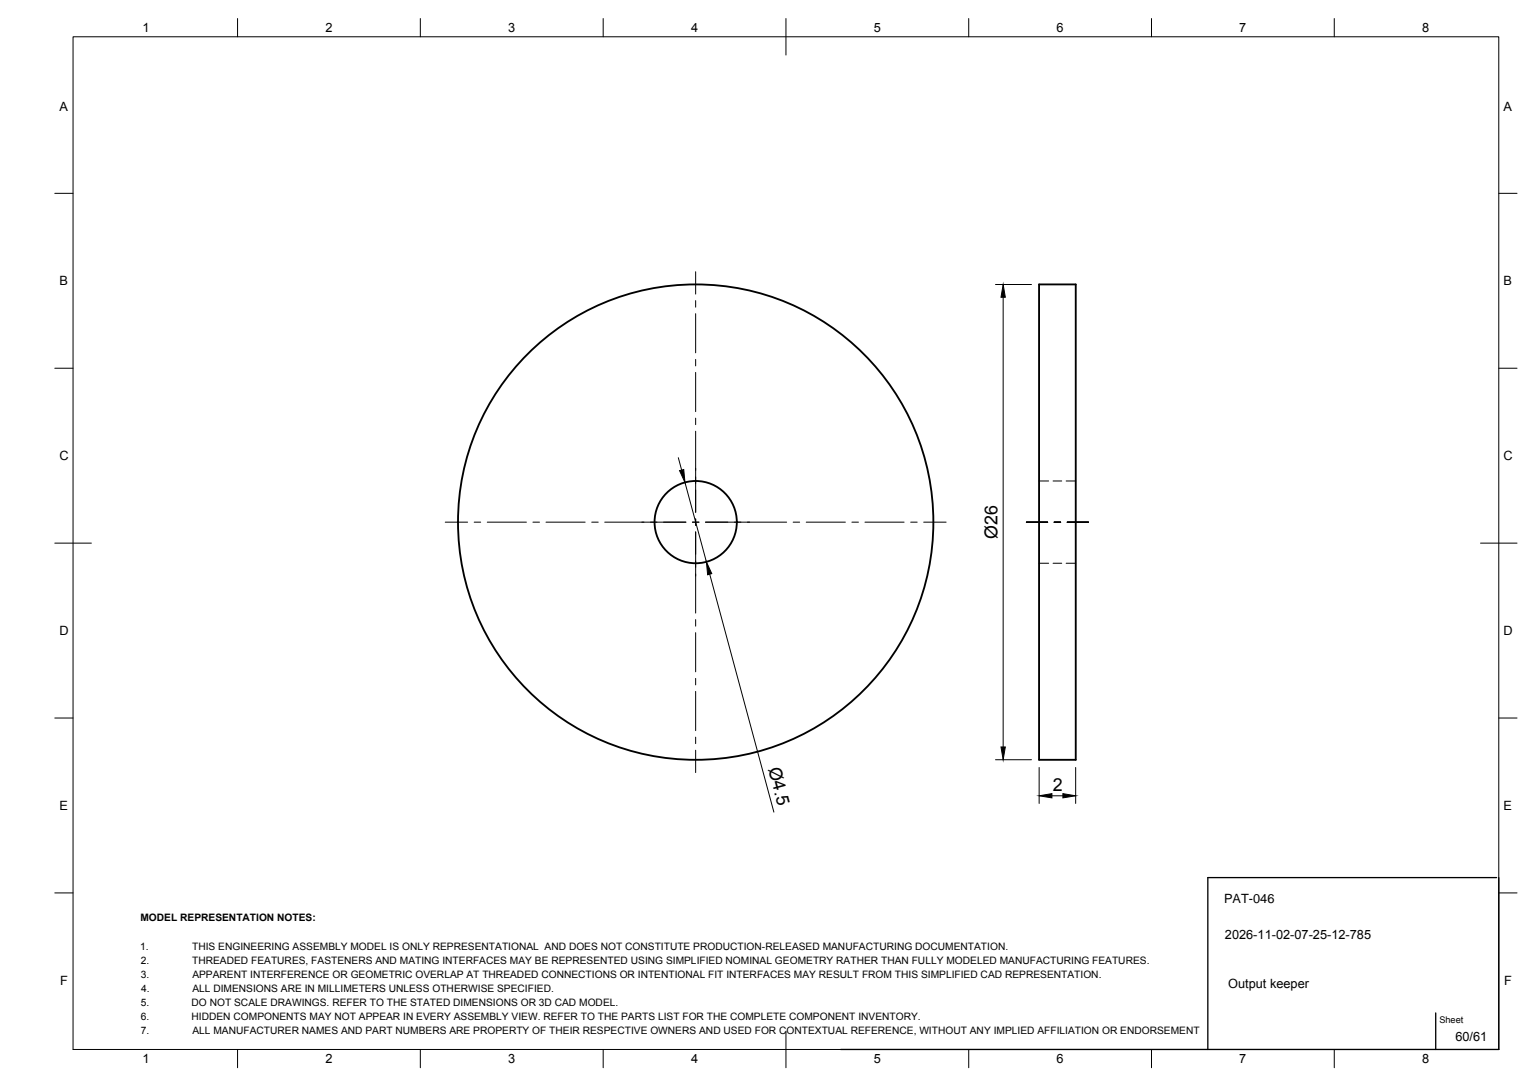
ISO-10303-21;
HEADER;
/* Generated by software containing ST-Developer
 * from STEP Tools, Inc. (www.steptools.com) 
 */

FILE_DESCRIPTION(
/* description */ ('Gear mesh backlash fixture'),
/* implementation_level */ '2;1');

FILE_NAME(
/* name */ 'Output keeper.step',
/* time_stamp */ '2026-10-28T03:26:00-07:00',
/* author */ (''),
/* organization */ (''),
/* preprocessor_version */ 'ST-DEVELOPER v20.2',
/* originating_system */ 'Autodesk Translation Framework v15.17.0.0',
/* authorisation */ '');

FILE_SCHEMA (('AUTOMOTIVE_DESIGN { 1 0 10303 214 3 1 1 }'));
ENDSEC;

DATA;
#10=MECHANICAL_DESIGN_GEOMETRIC_PRESENTATION_REPRESENTATION('',(#1077),#57900);
#962=SHAPE_REPRESENTATION_RELATIONSHIP('SRR','None',#58163,#1012);
#1012=ADVANCED_BREP_SHAPE_REPRESENTATION('',(#1140),#57896);
#1077=STYLED_ITEM('',(#58479),#1140);
#1140=MANIFOLD_SOLID_BREP('Body1',#13639);
#1323=FACE_BOUND('',#3208,.T.);
#1324=FACE_BOUND('',#3210,.T.);
#1626=PLANE('',#15289);
#1627=PLANE('',#15290);
#2260=FACE_OUTER_BOUND('',#3205,.T.);
#2261=FACE_OUTER_BOUND('',#3206,.T.);
#2262=FACE_OUTER_BOUND('',#3207,.T.);
#2263=FACE_OUTER_BOUND('',#3209,.T.);
#3205=EDGE_LOOP('',(#11477,#11478,#11479,#11480));
#3206=EDGE_LOOP('',(#11481,#11482,#11483,#11484));
#3207=EDGE_LOOP('',(#11485));
#3208=EDGE_LOOP('',(#11486));
#3209=EDGE_LOOP('',(#11487));
#3210=EDGE_LOOP('',(#11488));
#4084=LINE('',#34028,#4973);
#4085=LINE('',#34034,#4974);
#4973=VECTOR('',#18431,0.225);
#4974=VECTOR('',#18438,1.3);
#5683=CIRCLE('',#15284,0.225);
#5684=CIRCLE('',#15285,0.225);
#5685=CIRCLE('',#15287,1.3);
#5686=CIRCLE('',#15288,1.3);
#6658=VERTEX_POINT('',#34025);
#6659=VERTEX_POINT('',#34027);
#6660=VERTEX_POINT('',#34031);
#6661=VERTEX_POINT('',#34033);
#8325=EDGE_CURVE('',#6658,#6658,#5683,.T.);
#8326=EDGE_CURVE('',#6658,#6659,#4084,.T.);
#8327=EDGE_CURVE('',#6659,#6659,#5684,.T.);
#8328=EDGE_CURVE('',#6660,#6660,#5685,.T.);
#8329=EDGE_CURVE('',#6660,#6661,#4085,.T.);
#8330=EDGE_CURVE('',#6661,#6661,#5686,.T.);
#11477=ORIENTED_EDGE('',*,*,#8325,.F.);
#11478=ORIENTED_EDGE('',*,*,#8326,.T.);
#11479=ORIENTED_EDGE('',*,*,#8327,.T.);
#11480=ORIENTED_EDGE('',*,*,#8326,.F.);
#11481=ORIENTED_EDGE('',*,*,#8328,.F.);
#11482=ORIENTED_EDGE('',*,*,#8329,.T.);
#11483=ORIENTED_EDGE('',*,*,#8330,.T.);
#11484=ORIENTED_EDGE('',*,*,#8329,.F.);
#11485=ORIENTED_EDGE('',*,*,#8328,.T.);
#11486=ORIENTED_EDGE('',*,*,#8325,.T.);
#11487=ORIENTED_EDGE('',*,*,#8330,.F.);
#11488=ORIENTED_EDGE('',*,*,#8327,.F.);
#12764=CYLINDRICAL_SURFACE('',#15283,0.225);
#12765=CYLINDRICAL_SURFACE('',#15286,1.3);
#13377=ADVANCED_FACE('',(#2260),#12764,.F.);
#13378=ADVANCED_FACE('',(#2261),#12765,.T.);
#13379=ADVANCED_FACE('',(#2262,#1323),#1626,.T.);
#13380=ADVANCED_FACE('',(#2263,#1324),#1627,.F.);
#13639=CLOSED_SHELL('',(#13377,#13378,#13379,#13380));
#15282=AXIS2_PLACEMENT_3D('',#34023,#18425,#18426);
#15283=AXIS2_PLACEMENT_3D('',#34024,#18427,#18428);
#15284=AXIS2_PLACEMENT_3D('',#34026,#18429,#18430);
#15285=AXIS2_PLACEMENT_3D('',#34029,#18432,#18433);
#15286=AXIS2_PLACEMENT_3D('',#34030,#18434,#18435);
#15287=AXIS2_PLACEMENT_3D('',#34032,#18436,#18437);
#15288=AXIS2_PLACEMENT_3D('',#34035,#18439,#18440);
#15289=AXIS2_PLACEMENT_3D('',#34036,#18441,#18442);
#15290=AXIS2_PLACEMENT_3D('',#34037,#18443,#18444);
#18425=DIRECTION('axis',(0.,0.,1.));
#18426=DIRECTION('refdir',(1.,0.,0.));
#18427=DIRECTION('center_axis',(0.,0.,1.));
#18428=DIRECTION('ref_axis',(1.,0.,0.));
#18429=DIRECTION('center_axis',(0.,0.,-1.));
#18430=DIRECTION('ref_axis',(1.,0.,0.));
#18431=DIRECTION('',(0.,0.,-1.));
#18432=DIRECTION('center_axis',(0.,0.,-1.));
#18433=DIRECTION('ref_axis',(1.,0.,0.));
#18434=DIRECTION('center_axis',(0.,0.,1.));
#18435=DIRECTION('ref_axis',(1.,0.,0.));
#18436=DIRECTION('center_axis',(0.,0.,1.));
#18437=DIRECTION('ref_axis',(1.,0.,0.));
#18438=DIRECTION('',(0.,0.,-1.));
#18439=DIRECTION('center_axis',(0.,0.,1.));
#18440=DIRECTION('ref_axis',(1.,0.,0.));
#18441=DIRECTION('center_axis',(0.,0.,1.));
#18442=DIRECTION('ref_axis',(1.,0.,0.));
#18443=DIRECTION('center_axis',(0.,0.,1.));
#18444=DIRECTION('ref_axis',(1.,0.,0.));
#34023=CARTESIAN_POINT('',(0.,0.,0.));
#34024=CARTESIAN_POINT('Origin',(6.,0.,15.));
#34025=CARTESIAN_POINT('',(5.775,-2.75545529808154E-17,15.2));
#34026=CARTESIAN_POINT('Origin',(6.,0.,15.2));
#34027=CARTESIAN_POINT('',(5.775,-2.75545529808154E-17,15.));
#34028=CARTESIAN_POINT('',(5.775,-2.75545529808154E-17,15.));
#34029=CARTESIAN_POINT('Origin',(6.,0.,15.));
#34030=CARTESIAN_POINT('Origin',(6.,0.,15.));
#34031=CARTESIAN_POINT('',(4.7,-1.59204083889156E-16,15.2));
#34032=CARTESIAN_POINT('Origin',(6.,0.,15.2));
#34033=CARTESIAN_POINT('',(4.7,-1.59204083889156E-16,15.));
#34034=CARTESIAN_POINT('',(4.7,-1.59204083889156E-16,15.));
#34035=CARTESIAN_POINT('Origin',(6.,0.,15.));
#34036=CARTESIAN_POINT('Origin',(6.,0.,15.2));
#34037=CARTESIAN_POINT('Origin',(6.,0.,15.));
#57837=UNCERTAINTY_MEASURE_WITH_UNIT(LENGTH_MEASURE(0.001),#57901,
'DISTANCE_ACCURACY_VALUE',
'Maximum model space distance between geometric entities at asserted c
onnectivities');
#57841=UNCERTAINTY_MEASURE_WITH_UNIT(LENGTH_MEASURE(0.001),#57901,
'DISTANCE_ACCURACY_VALUE',
'Maximum model space distance between geometric entities at asserted c
onnectivities');
#57896=(
GEOMETRIC_REPRESENTATION_CONTEXT(3)
GLOBAL_UNCERTAINTY_ASSIGNED_CONTEXT((#57837))
GLOBAL_UNIT_ASSIGNED_CONTEXT((#57901,#57903,#57904))
REPRESENTATION_CONTEXT('','3D')
);
#57900=(
GEOMETRIC_REPRESENTATION_CONTEXT(3)
GLOBAL_UNCERTAINTY_ASSIGNED_CONTEXT((#57841))
GLOBAL_UNIT_ASSIGNED_CONTEXT((#57901,#57903,#57904))
REPRESENTATION_CONTEXT('','3D')
);
#57901=(
LENGTH_UNIT()
NAMED_UNIT(*)
SI_UNIT(.CENTI.,.METRE.)
);
#57903=(
NAMED_UNIT(*)
PLANE_ANGLE_UNIT()
SI_UNIT($,.RADIAN.)
);
#57904=(
NAMED_UNIT(*)
SI_UNIT($,.STERADIAN.)
SOLID_ANGLE_UNIT()
);
#57959=SHAPE_DEFINITION_REPRESENTATION(#58030,#58163);
#58030=PRODUCT_DEFINITION_SHAPE('',$,#58222);
#58163=SHAPE_REPRESENTATION('',(#15282),#57896);
#58167=PRODUCT_DEFINITION_CONTEXT('part definition',#58343,'design');
#58222=PRODUCT_DEFINITION('Output keeper','Output keeper',#58280,#58167);
#58280=PRODUCT_DEFINITION_FORMATION('',$,#58399);
#58343=APPLICATION_CONTEXT(
'Core Data for Automotive Mechanical Design Process');
#58344=PRODUCT_CONTEXT('part definition',#58343,'mechanical');
#58399=PRODUCT('Output keeper','Output keeper','Output keeper',(#58344));
#58473=COLOUR_RGB('Off White',0.89,0.88,0.83);
#58474=FILL_AREA_STYLE_COLOUR('',#58473);
#58475=FILL_AREA_STYLE('',(#58474));
#58476=SURFACE_STYLE_FILL_AREA(#58475);
#58477=SURFACE_SIDE_STYLE('',(#58476));
#58478=SURFACE_STYLE_USAGE(.BOTH.,#58477);
#58479=PRESENTATION_STYLE_ASSIGNMENT((#58478));
ENDSEC;
END-ISO-10303-21;
